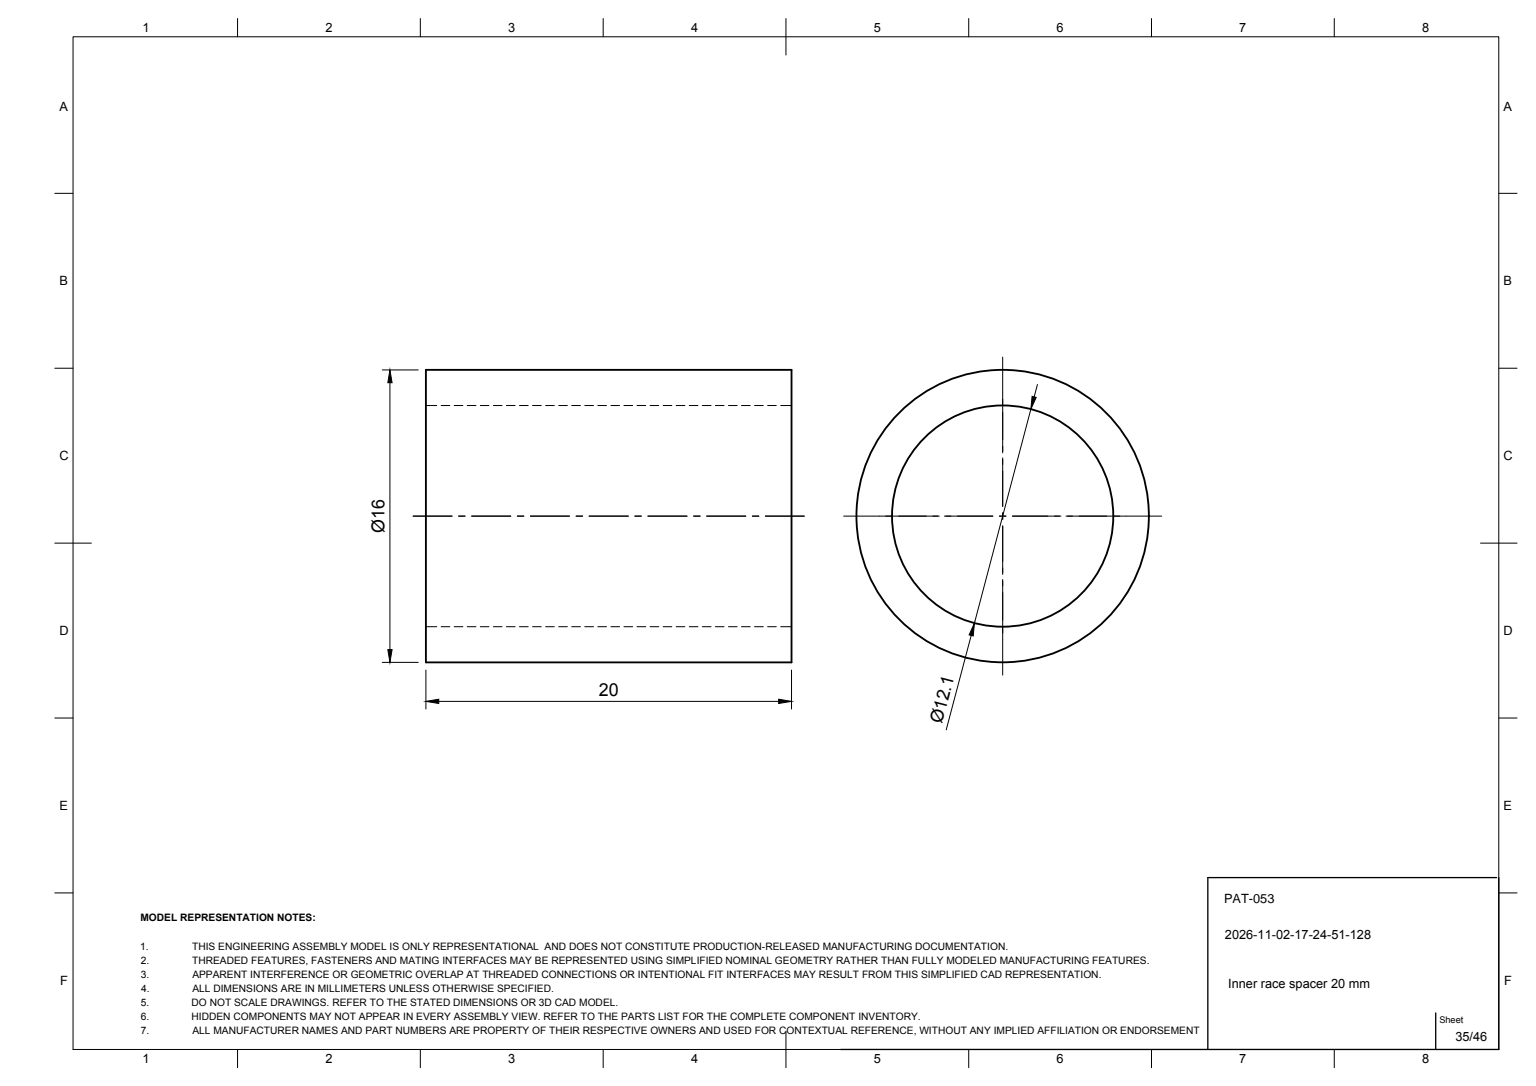
ISO-10303-21;
HEADER;
/* Generated by software containing ST-Developer
 * from STEP Tools, Inc. (www.steptools.com) 
 */

FILE_DESCRIPTION(
/* description */ ('Hand-operated arbor press'),
/* implementation_level */ '2;1');

FILE_NAME(
/* name */ 'Inner race spacer 20 mm.step',
/* time_stamp */ '2026-10-28T03:25:25-07:00',
/* author */ (''),
/* organization */ (''),
/* preprocessor_version */ 'ST-DEVELOPER v20.2',
/* originating_system */ 'Autodesk Translation Framework v15.17.0.0',
/* authorisation */ '');

FILE_SCHEMA (('AUTOMOTIVE_DESIGN { 1 0 10303 214 3 1 1 }'));
ENDSEC;

DATA;
#10=MECHANICAL_DESIGN_GEOMETRIC_PRESENTATION_REPRESENTATION('',(#620),#32751);
#529=SHAPE_REPRESENTATION_RELATIONSHIP('SRR','None',#32961,#571);
#571=ADVANCED_BREP_SHAPE_REPRESENTATION('',(#667),#32735);
#620=STYLED_ITEM('',(#33242),#667);
#667=MANIFOLD_SOLID_BREP('Body1',#12519);
#821=FACE_BOUND('',#2616,.T.);
#822=FACE_BOUND('',#2618,.T.);
#1206=PLANE('',#13829);
#1207=PLANE('',#13830);
#1791=FACE_OUTER_BOUND('',#2613,.T.);
#1792=FACE_OUTER_BOUND('',#2614,.T.);
#1793=FACE_OUTER_BOUND('',#2615,.T.);
#1794=FACE_OUTER_BOUND('',#2617,.T.);
#2613=EDGE_LOOP('',(#10788,#10789,#10790,#10791));
#2614=EDGE_LOOP('',(#10792,#10793,#10794,#10795));
#2615=EDGE_LOOP('',(#10796));
#2616=EDGE_LOOP('',(#10797));
#2617=EDGE_LOOP('',(#10798));
#2618=EDGE_LOOP('',(#10799));
#3754=LINE('',#20603,#4925);
#3755=LINE('',#20609,#4926);
#4925=VECTOR('',#16737,0.605);
#4926=VECTOR('',#16744,0.8);
#5450=CIRCLE('',#13824,0.605);
#5451=CIRCLE('',#13825,0.605);
#5452=CIRCLE('',#13827,0.8);
#5453=CIRCLE('',#13828,0.8);
#6383=VERTEX_POINT('',#20600);
#6384=VERTEX_POINT('',#20602);
#6385=VERTEX_POINT('',#20606);
#6386=VERTEX_POINT('',#20608);
#7897=EDGE_CURVE('',#6383,#6383,#5450,.T.);
#7898=EDGE_CURVE('',#6383,#6384,#3754,.T.);
#7899=EDGE_CURVE('',#6384,#6384,#5451,.T.);
#7900=EDGE_CURVE('',#6385,#6385,#5452,.T.);
#7901=EDGE_CURVE('',#6385,#6386,#3755,.T.);
#7902=EDGE_CURVE('',#6386,#6386,#5453,.T.);
#10788=ORIENTED_EDGE('',*,*,#7897,.F.);
#10789=ORIENTED_EDGE('',*,*,#7898,.T.);
#10790=ORIENTED_EDGE('',*,*,#7899,.T.);
#10791=ORIENTED_EDGE('',*,*,#7898,.F.);
#10792=ORIENTED_EDGE('',*,*,#7900,.F.);
#10793=ORIENTED_EDGE('',*,*,#7901,.T.);
#10794=ORIENTED_EDGE('',*,*,#7902,.T.);
#10795=ORIENTED_EDGE('',*,*,#7901,.F.);
#10796=ORIENTED_EDGE('',*,*,#7900,.T.);
#10797=ORIENTED_EDGE('',*,*,#7897,.T.);
#10798=ORIENTED_EDGE('',*,*,#7902,.F.);
#10799=ORIENTED_EDGE('',*,*,#7899,.F.);
#11754=CYLINDRICAL_SURFACE('',#13823,0.605);
#11755=CYLINDRICAL_SURFACE('',#13826,0.8);
#12300=ADVANCED_FACE('',(#1791),#11754,.F.);
#12301=ADVANCED_FACE('',(#1792),#11755,.T.);
#12302=ADVANCED_FACE('',(#1793,#821),#1206,.T.);
#12303=ADVANCED_FACE('',(#1794,#822),#1207,.F.);
#12519=CLOSED_SHELL('',(#12300,#12301,#12302,#12303));
#13822=AXIS2_PLACEMENT_3D('',#20598,#16731,#16732);
#13823=AXIS2_PLACEMENT_3D('',#20599,#16733,#16734);
#13824=AXIS2_PLACEMENT_3D('',#20601,#16735,#16736);
#13825=AXIS2_PLACEMENT_3D('',#20604,#16738,#16739);
#13826=AXIS2_PLACEMENT_3D('',#20605,#16740,#16741);
#13827=AXIS2_PLACEMENT_3D('',#20607,#16742,#16743);
#13828=AXIS2_PLACEMENT_3D('',#20610,#16745,#16746);
#13829=AXIS2_PLACEMENT_3D('',#20611,#16747,#16748);
#13830=AXIS2_PLACEMENT_3D('',#20612,#16749,#16750);
#16731=DIRECTION('axis',(0.,0.,1.));
#16732=DIRECTION('refdir',(1.,0.,0.));
#16733=DIRECTION('center_axis',(0.,1.,0.));
#16734=DIRECTION('ref_axis',(1.,0.,0.));
#16735=DIRECTION('center_axis',(0.,-1.,0.));
#16736=DIRECTION('ref_axis',(1.,0.,0.));
#16737=DIRECTION('',(0.,-1.,0.));
#16738=DIRECTION('center_axis',(0.,-1.,0.));
#16739=DIRECTION('ref_axis',(1.,0.,0.));
#16740=DIRECTION('center_axis',(0.,1.,0.));
#16741=DIRECTION('ref_axis',(1.,0.,0.));
#16742=DIRECTION('center_axis',(0.,1.,0.));
#16743=DIRECTION('ref_axis',(1.,0.,0.));
#16744=DIRECTION('',(0.,-1.,0.));
#16745=DIRECTION('center_axis',(0.,1.,0.));
#16746=DIRECTION('ref_axis',(1.,0.,0.));
#16747=DIRECTION('center_axis',(0.,1.,0.));
#16748=DIRECTION('ref_axis',(1.,0.,0.));
#16749=DIRECTION('center_axis',(0.,1.,0.));
#16750=DIRECTION('ref_axis',(1.,0.,0.));
#20598=CARTESIAN_POINT('',(0.,0.,0.));
#20599=CARTESIAN_POINT('Origin',(-3.25,-5.5,20.));
#20600=CARTESIAN_POINT('',(-3.855,-3.5,20.));
#20601=CARTESIAN_POINT('Origin',(-3.25,-3.5,20.));
#20602=CARTESIAN_POINT('',(-3.855,-5.5,20.));
#20603=CARTESIAN_POINT('',(-3.855,-5.5,20.));
#20604=CARTESIAN_POINT('Origin',(-3.25,-5.5,20.));
#20605=CARTESIAN_POINT('Origin',(-3.25,-5.5,20.));
#20606=CARTESIAN_POINT('',(-4.05,-3.5,20.));
#20607=CARTESIAN_POINT('Origin',(-3.25,-3.5,20.));
#20608=CARTESIAN_POINT('',(-4.05,-5.5,20.));
#20609=CARTESIAN_POINT('',(-4.05,-5.5,20.));
#20610=CARTESIAN_POINT('Origin',(-3.25,-5.5,20.));
#20611=CARTESIAN_POINT('Origin',(-3.25,-3.5,20.));
#20612=CARTESIAN_POINT('Origin',(-3.25,-5.5,20.));
#32686=UNCERTAINTY_MEASURE_WITH_UNIT(LENGTH_MEASURE(0.001),#32752,
'DISTANCE_ACCURACY_VALUE',
'Maximum model space distance between geometric entities at asserted c
onnectivities');
#32702=UNCERTAINTY_MEASURE_WITH_UNIT(LENGTH_MEASURE(0.001),#32752,
'DISTANCE_ACCURACY_VALUE',
'Maximum model space distance between geometric entities at asserted c
onnectivities');
#32735=(
GEOMETRIC_REPRESENTATION_CONTEXT(3)
GLOBAL_UNCERTAINTY_ASSIGNED_CONTEXT((#32686))
GLOBAL_UNIT_ASSIGNED_CONTEXT((#32752,#32754,#32755))
REPRESENTATION_CONTEXT('','3D')
);
#32751=(
GEOMETRIC_REPRESENTATION_CONTEXT(3)
GLOBAL_UNCERTAINTY_ASSIGNED_CONTEXT((#32702))
GLOBAL_UNIT_ASSIGNED_CONTEXT((#32752,#32754,#32755))
REPRESENTATION_CONTEXT('','3D')
);
#32752=(
LENGTH_UNIT()
NAMED_UNIT(*)
SI_UNIT(.CENTI.,.METRE.)
);
#32754=(
NAMED_UNIT(*)
PLANE_ANGLE_UNIT()
SI_UNIT($,.RADIAN.)
);
#32755=(
NAMED_UNIT(*)
SI_UNIT($,.STERADIAN.)
SOLID_ANGLE_UNIT()
);
#32788=SHAPE_DEFINITION_REPRESENTATION(#32845,#32961);
#32845=PRODUCT_DEFINITION_SHAPE('',$,#33010);
#32961=SHAPE_REPRESENTATION('',(#13822),#32735);
#32977=PRODUCT_DEFINITION_CONTEXT('part definition',#33123,'design');
#33010=PRODUCT_DEFINITION('Inner race spacer 20 mm',
'Inner race spacer 20 mm',#33058,#32977);
#33058=PRODUCT_DEFINITION_FORMATION('',$,#33157);
#33123=APPLICATION_CONTEXT(
'Core Data for Automotive Mechanical Design Process');
#33124=PRODUCT_CONTEXT('part definition',#33123,'mechanical');
#33157=PRODUCT('Inner race spacer 20 mm','Inner race spacer 20 mm',
'Inner race spacer 20 mm',(#33124));
#33236=COLOUR_RGB('Grey',0.48,0.52,0.57);
#33237=FILL_AREA_STYLE_COLOUR('',#33236);
#33238=FILL_AREA_STYLE('',(#33237));
#33239=SURFACE_STYLE_FILL_AREA(#33238);
#33240=SURFACE_SIDE_STYLE('',(#33239));
#33241=SURFACE_STYLE_USAGE(.BOTH.,#33240);
#33242=PRESENTATION_STYLE_ASSIGNMENT((#33241));
ENDSEC;
END-ISO-10303-21;
